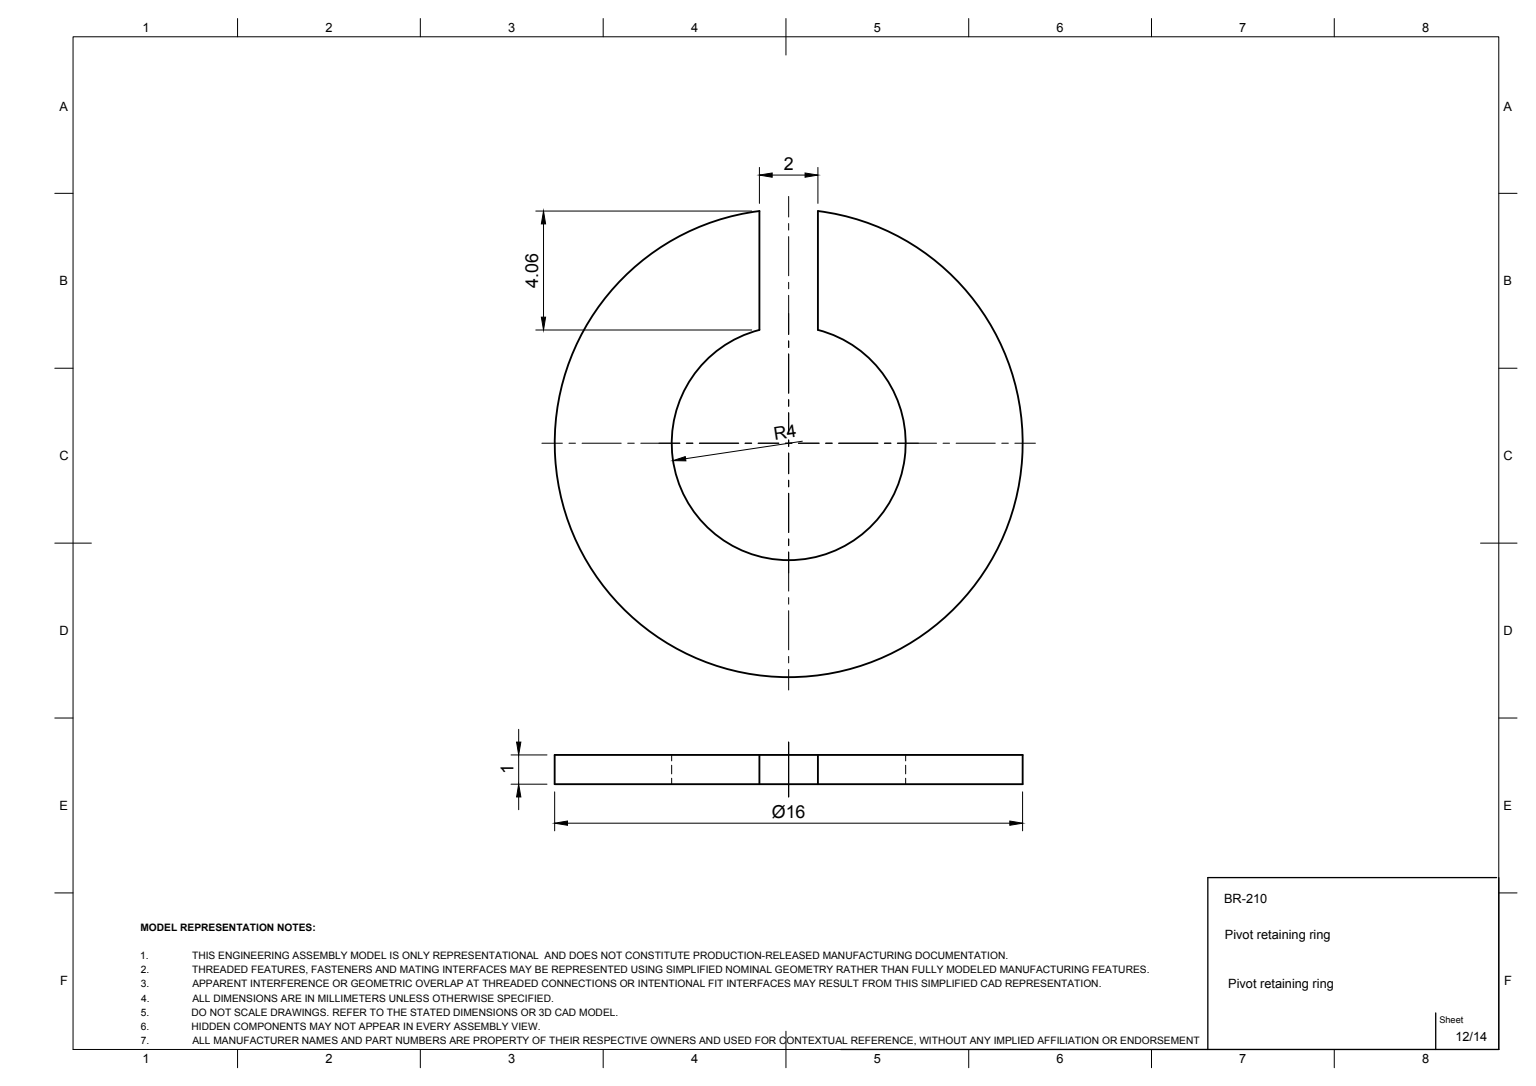
ISO-10303-21;
HEADER;
/* Generated by software containing ST-Developer
 * from STEP Tools, Inc. (www.steptools.com) 
 */

FILE_DESCRIPTION(
/* description */ ('Independent 1:2 reduction pantograph. 120 mm parallelogram sides; fix
ed fulcrum on the extension of a 240 mm link. Drawing point halfway al
ong its link, so its XY displacement is one half of the tracing point.
 Replaceable pivot bushes and retained pins. Calibration and productio
n accuracy unassigned.'),
/* implementation_level */ '2;1');

FILE_NAME(
/* name */ 'Pivot retaining ring.step',
/* time_stamp */ '2026-11-07T22:11:57-08:00',
/* author */ (''),
/* organization */ (''),
/* preprocessor_version */ 'ST-DEVELOPER v20.2',
/* originating_system */ 'Autodesk Translation Framework v15.17.0.0',
/* authorisation */ '');

FILE_SCHEMA (('AUTOMOTIVE_DESIGN { 1 0 10303 214 3 1 1 }'));
ENDSEC;

DATA;
#10=MECHANICAL_DESIGN_GEOMETRIC_PRESENTATION_REPRESENTATION('',(#197),#2926);
#171=SHAPE_REPRESENTATION_RELATIONSHIP('SRR','None',#3008,#184);
#184=ADVANCED_BREP_SHAPE_REPRESENTATION('',(#210),#2924);
#197=STYLED_ITEM('',(#3080),#210);
#210=MANIFOLD_SOLID_BREP('Body1',#1552);
#300=PLANE('',#1876);
#301=PLANE('',#1877);
#302=PLANE('',#1878);
#303=PLANE('',#1885);
#388=FACE_OUTER_BOUND('',#526,.T.);
#389=FACE_OUTER_BOUND('',#527,.T.);
#390=FACE_OUTER_BOUND('',#528,.T.);
#391=FACE_OUTER_BOUND('',#529,.T.);
#392=FACE_OUTER_BOUND('',#530,.T.);
#393=FACE_OUTER_BOUND('',#531,.T.);
#526=EDGE_LOOP('',(#1373,#1374,#1375,#1376));
#527=EDGE_LOOP('',(#1377,#1378,#1379,#1380));
#528=EDGE_LOOP('',(#1381,#1382,#1383,#1384));
#529=EDGE_LOOP('',(#1385,#1386,#1387,#1388));
#530=EDGE_LOOP('',(#1389,#1390,#1391,#1392));
#531=EDGE_LOOP('',(#1393,#1394,#1395,#1396));
#606=LINE('',#2826,#687);
#607=LINE('',#2828,#688);
#608=LINE('',#2830,#689);
#609=LINE('',#2831,#690);
#610=LINE('',#2835,#691);
#611=LINE('',#2837,#692);
#612=LINE('',#2839,#693);
#613=LINE('',#2840,#694);
#687=VECTOR('',#2358,10.);
#688=VECTOR('',#2359,10.);
#689=VECTOR('',#2360,10.);
#690=VECTOR('',#2361,10.);
#691=VECTOR('',#2364,10.);
#692=VECTOR('',#2365,10.);
#693=VECTOR('',#2366,10.);
#694=VECTOR('',#2367,10.);
#779=CIRCLE('',#1879,8.);
#780=CIRCLE('',#1880,4.);
#781=CIRCLE('',#1882,4.);
#782=CIRCLE('',#1884,8.);
#887=VERTEX_POINT('',#2824);
#888=VERTEX_POINT('',#2825);
#889=VERTEX_POINT('',#2827);
#890=VERTEX_POINT('',#2829);
#891=VERTEX_POINT('',#2833);
#892=VERTEX_POINT('',#2834);
#893=VERTEX_POINT('',#2836);
#894=VERTEX_POINT('',#2838);
#1051=EDGE_CURVE('',#887,#888,#606,.T.);
#1052=EDGE_CURVE('',#889,#887,#607,.T.);
#1053=EDGE_CURVE('',#890,#889,#608,.T.);
#1054=EDGE_CURVE('',#888,#890,#609,.T.);
#1055=EDGE_CURVE('',#891,#892,#610,.T.);
#1056=EDGE_CURVE('',#893,#891,#611,.T.);
#1057=EDGE_CURVE('',#894,#893,#612,.T.);
#1058=EDGE_CURVE('',#892,#894,#613,.T.);
#1059=EDGE_CURVE('',#889,#894,#779,.T.);
#1060=EDGE_CURVE('',#892,#887,#780,.T.);
#1061=EDGE_CURVE('',#891,#888,#781,.T.);
#1062=EDGE_CURVE('',#890,#893,#782,.T.);
#1373=ORIENTED_EDGE('',*,*,#1051,.F.);
#1374=ORIENTED_EDGE('',*,*,#1052,.F.);
#1375=ORIENTED_EDGE('',*,*,#1053,.F.);
#1376=ORIENTED_EDGE('',*,*,#1054,.F.);
#1377=ORIENTED_EDGE('',*,*,#1055,.F.);
#1378=ORIENTED_EDGE('',*,*,#1056,.F.);
#1379=ORIENTED_EDGE('',*,*,#1057,.F.);
#1380=ORIENTED_EDGE('',*,*,#1058,.F.);
#1381=ORIENTED_EDGE('',*,*,#1058,.T.);
#1382=ORIENTED_EDGE('',*,*,#1059,.F.);
#1383=ORIENTED_EDGE('',*,*,#1052,.T.);
#1384=ORIENTED_EDGE('',*,*,#1060,.F.);
#1385=ORIENTED_EDGE('',*,*,#1055,.T.);
#1386=ORIENTED_EDGE('',*,*,#1060,.T.);
#1387=ORIENTED_EDGE('',*,*,#1051,.T.);
#1388=ORIENTED_EDGE('',*,*,#1061,.F.);
#1389=ORIENTED_EDGE('',*,*,#1057,.T.);
#1390=ORIENTED_EDGE('',*,*,#1062,.F.);
#1391=ORIENTED_EDGE('',*,*,#1053,.T.);
#1392=ORIENTED_EDGE('',*,*,#1059,.T.);
#1393=ORIENTED_EDGE('',*,*,#1056,.T.);
#1394=ORIENTED_EDGE('',*,*,#1061,.T.);
#1395=ORIENTED_EDGE('',*,*,#1054,.T.);
#1396=ORIENTED_EDGE('',*,*,#1062,.T.);
#1446=CYLINDRICAL_SURFACE('',#1881,4.);
#1447=CYLINDRICAL_SURFACE('',#1883,8.);
#1532=ADVANCED_FACE('',(#388),#300,.F.);
#1533=ADVANCED_FACE('',(#389),#301,.F.);
#1534=ADVANCED_FACE('',(#390),#302,.F.);
#1535=ADVANCED_FACE('',(#391),#1446,.F.);
#1536=ADVANCED_FACE('',(#392),#1447,.T.);
#1537=ADVANCED_FACE('',(#393),#303,.T.);
#1552=CLOSED_SHELL('',(#1532,#1533,#1534,#1535,#1536,#1537));
#1875=AXIS2_PLACEMENT_3D('',#2822,#2354,#2355);
#1876=AXIS2_PLACEMENT_3D('',#2823,#2356,#2357);
#1877=AXIS2_PLACEMENT_3D('',#2832,#2362,#2363);
#1878=AXIS2_PLACEMENT_3D('',#2841,#2368,#2369);
#1879=AXIS2_PLACEMENT_3D('',#2842,#2370,#2371);
#1880=AXIS2_PLACEMENT_3D('',#2843,#2372,#2373);
#1881=AXIS2_PLACEMENT_3D('',#2844,#2374,#2375);
#1882=AXIS2_PLACEMENT_3D('',#2845,#2376,#2377);
#1883=AXIS2_PLACEMENT_3D('',#2846,#2378,#2379);
#1884=AXIS2_PLACEMENT_3D('',#2847,#2380,#2381);
#1885=AXIS2_PLACEMENT_3D('',#2848,#2382,#2383);
#2354=DIRECTION('axis',(0.,0.,1.));
#2355=DIRECTION('refdir',(1.,0.,0.));
#2356=DIRECTION('center_axis',(-1.,0.,0.));
#2357=DIRECTION('ref_axis',(0.,1.,0.));
#2358=DIRECTION('',(0.,0.,1.));
#2359=DIRECTION('',(0.,-1.,0.));
#2360=DIRECTION('',(0.,0.,-1.));
#2361=DIRECTION('',(0.,1.,0.));
#2362=DIRECTION('center_axis',(1.,0.,0.));
#2363=DIRECTION('ref_axis',(0.,-1.,0.));
#2364=DIRECTION('',(0.,0.,-1.));
#2365=DIRECTION('',(0.,-1.,0.));
#2366=DIRECTION('',(0.,0.,1.));
#2367=DIRECTION('',(0.,1.,0.));
#2368=DIRECTION('center_axis',(0.,0.,1.));
#2369=DIRECTION('ref_axis',(1.,0.,0.));
#2370=DIRECTION('center_axis',(0.,0.,1.));
#2371=DIRECTION('ref_axis',(1.,0.,0.));
#2372=DIRECTION('center_axis',(0.,0.,-1.));
#2373=DIRECTION('ref_axis',(1.,0.,0.));
#2374=DIRECTION('center_axis',(0.,0.,1.));
#2375=DIRECTION('ref_axis',(6.12323399573677E-17,-1.,0.));
#2376=DIRECTION('center_axis',(0.,0.,-1.));
#2377=DIRECTION('ref_axis',(1.,0.,0.));
#2378=DIRECTION('center_axis',(0.,0.,1.));
#2379=DIRECTION('ref_axis',(6.12323399573677E-17,-1.,0.));
#2380=DIRECTION('center_axis',(0.,0.,1.));
#2381=DIRECTION('ref_axis',(1.,0.,0.));
#2382=DIRECTION('center_axis',(0.,0.,1.));
#2383=DIRECTION('ref_axis',(1.,0.,0.));
#2822=CARTESIAN_POINT('',(0.,0.,0.));
#2823=CARTESIAN_POINT('Origin',(-1.,0.,1.));
#2824=CARTESIAN_POINT('',(-1.,3.87298334620742,0.));
#2825=CARTESIAN_POINT('',(-1.,3.87298334620742,1.));
#2826=CARTESIAN_POINT('',(-1.,3.87298334620742,0.));
#2827=CARTESIAN_POINT('',(-1.,7.93725393319377,0.));
#2828=CARTESIAN_POINT('',(-1.,0.,0.));
#2829=CARTESIAN_POINT('',(-1.,7.93725393319377,1.));
#2830=CARTESIAN_POINT('',(-1.,7.93725393319377,0.));
#2831=CARTESIAN_POINT('',(-1.,0.,1.));
#2832=CARTESIAN_POINT('Origin',(1.,16.,1.));
#2833=CARTESIAN_POINT('',(1.,3.87298334620742,1.));
#2834=CARTESIAN_POINT('',(1.,3.87298334620742,0.));
#2835=CARTESIAN_POINT('',(1.,3.87298334620742,0.));
#2836=CARTESIAN_POINT('',(1.,7.93725393319377,1.));
#2837=CARTESIAN_POINT('',(1.,8.,1.));
#2838=CARTESIAN_POINT('',(1.,7.93725393319377,0.));
#2839=CARTESIAN_POINT('',(1.,7.93725393319377,0.));
#2840=CARTESIAN_POINT('',(1.,8.,0.));
#2841=CARTESIAN_POINT('Origin',(0.,0.,0.));
#2842=CARTESIAN_POINT('Origin',(0.,0.,0.));
#2843=CARTESIAN_POINT('Origin',(0.,0.,0.));
#2844=CARTESIAN_POINT('Origin',(0.,0.,0.));
#2845=CARTESIAN_POINT('Origin',(0.,0.,1.));
#2846=CARTESIAN_POINT('Origin',(0.,0.,0.));
#2847=CARTESIAN_POINT('Origin',(0.,0.,1.));
#2848=CARTESIAN_POINT('Origin',(0.,0.,1.));
#2909=UNCERTAINTY_MEASURE_WITH_UNIT(LENGTH_MEASURE(0.01),#2927,
'DISTANCE_ACCURACY_VALUE',
'Maximum model space distance between geometric entities at asserted c
onnectivities');
#2911=UNCERTAINTY_MEASURE_WITH_UNIT(LENGTH_MEASURE(0.01),#2927,
'DISTANCE_ACCURACY_VALUE',
'Maximum model space distance between geometric entities at asserted c
onnectivities');
#2924=(
GEOMETRIC_REPRESENTATION_CONTEXT(3)
GLOBAL_UNCERTAINTY_ASSIGNED_CONTEXT((#2909))
GLOBAL_UNIT_ASSIGNED_CONTEXT((#2927,#2929,#2930))
REPRESENTATION_CONTEXT('','3D')
);
#2926=(
GEOMETRIC_REPRESENTATION_CONTEXT(3)
GLOBAL_UNCERTAINTY_ASSIGNED_CONTEXT((#2911))
GLOBAL_UNIT_ASSIGNED_CONTEXT((#2927,#2929,#2930))
REPRESENTATION_CONTEXT('','3D')
);
#2927=(
LENGTH_UNIT()
NAMED_UNIT(*)
SI_UNIT(.MILLI.,.METRE.)
);
#2929=(
NAMED_UNIT(*)
PLANE_ANGLE_UNIT()
SI_UNIT($,.RADIAN.)
);
#2930=(
NAMED_UNIT(*)
SI_UNIT($,.STERADIAN.)
SOLID_ANGLE_UNIT()
);
#2943=SHAPE_DEFINITION_REPRESENTATION(#2957,#3008);
#2957=PRODUCT_DEFINITION_SHAPE('',$,#3023);
#3008=SHAPE_REPRESENTATION('',(#1875),#2924);
#3010=PRODUCT_DEFINITION_CONTEXT('part definition',#3054,'design');
#3023=PRODUCT_DEFINITION('Pivot retaining ring','Pivot retaining ring',
#3037,#3010);
#3037=PRODUCT_DEFINITION_FORMATION('',$,#3068);
#3054=APPLICATION_CONTEXT(
'Core Data for Automotive Mechanical Design Process');
#3055=PRODUCT_CONTEXT('part definition',#3054,'mechanical');
#3068=PRODUCT('Pivot retaining ring','Pivot retaining ring',$,(#3055));
#3080=PRESENTATION_STYLE_ASSIGNMENT((#3092));
#3092=SURFACE_STYLE_USAGE(.BOTH.,#3104);
#3104=SURFACE_SIDE_STYLE('',(#3116));
#3116=SURFACE_STYLE_FILL_AREA(#3128);
#3128=FILL_AREA_STYLE('Dark gray',(#3140));
#3140=FILL_AREA_STYLE_COLOUR('Dark gray',#3152);
#3152=COLOUR_RGB('Dark gray',0.250980392156863,0.282352941176471,0.32156862745098);
ENDSEC;
END-ISO-10303-21;
